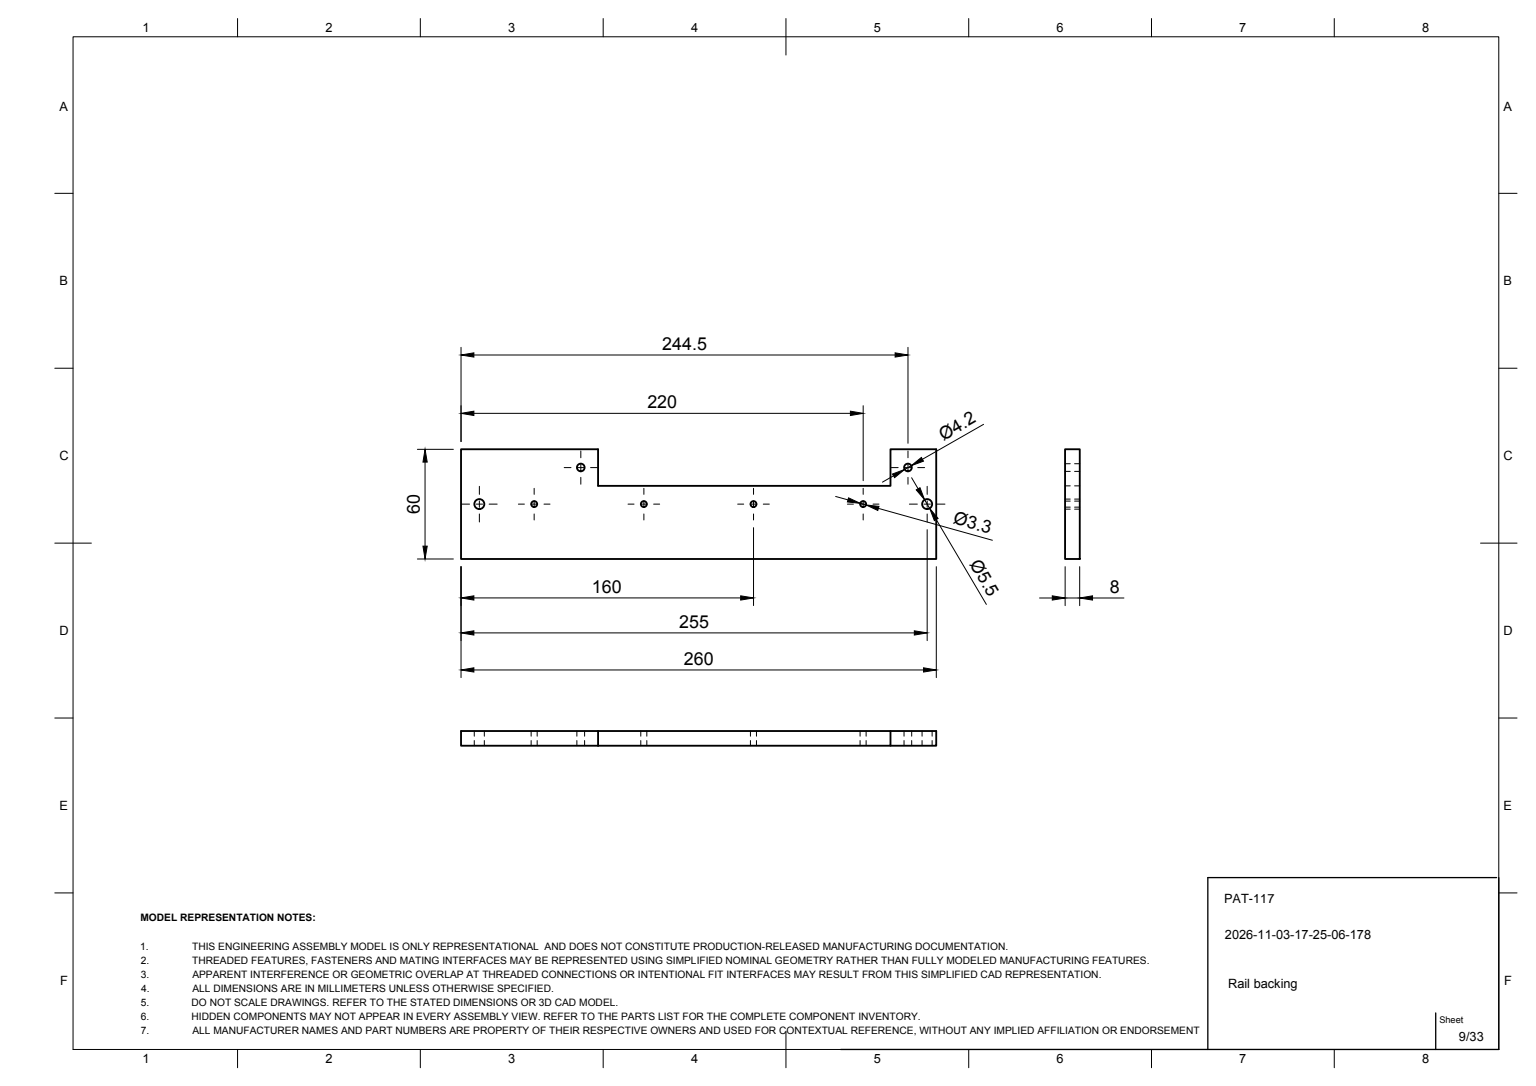
ISO-10303-21;
HEADER;
/* Generated by software containing ST-Developer
 * from STEP Tools, Inc. (www.steptools.com) 
 */

FILE_DESCRIPTION(
/* description */ ('Counterbalanced vertical column'),
/* implementation_level */ '2;1');

FILE_NAME(
/* name */ 'Rail backing.step',
/* time_stamp */ '2026-10-29T16:47:22-07:00',
/* author */ (''),
/* organization */ (''),
/* preprocessor_version */ 'ST-DEVELOPER v20.2',
/* originating_system */ 'Autodesk Translation Framework v15.17.0.0',
/* authorisation */ '');

FILE_SCHEMA (('AUTOMOTIVE_DESIGN { 1 0 10303 214 3 1 1 }'));
ENDSEC;

DATA;
#10=MECHANICAL_DESIGN_GEOMETRIC_PRESENTATION_REPRESENTATION('',(#354),#15040);
#284=SHAPE_REPRESENTATION_RELATIONSHIP('SRR','None',#15188,#319);
#319=ADVANCED_BREP_SHAPE_REPRESENTATION('',(#389),#15007);
#354=STYLED_ITEM('',(#15443),#389);
#389=MANIFOLD_SOLID_BREP('Body1',#7077);
#424=FACE_BOUND('',#1285,.T.);
#425=FACE_BOUND('',#1286,.T.);
#426=FACE_BOUND('',#1287,.T.);
#427=FACE_BOUND('',#1288,.T.);
#428=FACE_BOUND('',#1289,.T.);
#429=FACE_BOUND('',#1290,.T.);
#430=FACE_BOUND('',#1291,.T.);
#431=FACE_BOUND('',#1292,.T.);
#432=FACE_BOUND('',#1296,.T.);
#433=FACE_BOUND('',#1297,.T.);
#434=FACE_BOUND('',#1298,.T.);
#435=FACE_BOUND('',#1299,.T.);
#436=FACE_BOUND('',#1300,.T.);
#437=FACE_BOUND('',#1301,.T.);
#438=FACE_BOUND('',#1302,.T.);
#439=FACE_BOUND('',#1303,.T.);
#559=PLANE('',#7575);
#560=PLANE('',#7576);
#561=PLANE('',#7577);
#562=PLANE('',#7578);
#563=PLANE('',#7579);
#564=PLANE('',#7580);
#565=PLANE('',#7581);
#566=PLANE('',#7582);
#567=PLANE('',#7583);
#568=PLANE('',#7584);
#860=FACE_OUTER_BOUND('',#1273,.T.);
#861=FACE_OUTER_BOUND('',#1274,.T.);
#862=FACE_OUTER_BOUND('',#1275,.T.);
#863=FACE_OUTER_BOUND('',#1276,.T.);
#864=FACE_OUTER_BOUND('',#1277,.T.);
#865=FACE_OUTER_BOUND('',#1278,.T.);
#866=FACE_OUTER_BOUND('',#1279,.T.);
#867=FACE_OUTER_BOUND('',#1280,.T.);
#868=FACE_OUTER_BOUND('',#1281,.T.);
#869=FACE_OUTER_BOUND('',#1282,.T.);
#870=FACE_OUTER_BOUND('',#1283,.T.);
#871=FACE_OUTER_BOUND('',#1284,.T.);
#872=FACE_OUTER_BOUND('',#1293,.T.);
#873=FACE_OUTER_BOUND('',#1294,.T.);
#874=FACE_OUTER_BOUND('',#1295,.T.);
#875=FACE_OUTER_BOUND('',#1304,.T.);
#876=FACE_OUTER_BOUND('',#1305,.T.);
#877=FACE_OUTER_BOUND('',#1306,.T.);
#1273=EDGE_LOOP('',(#4920,#4921,#4922,#4923));
#1274=EDGE_LOOP('',(#4924,#4925,#4926,#4927));
#1275=EDGE_LOOP('',(#4928,#4929,#4930,#4931));
#1276=EDGE_LOOP('',(#4932,#4933,#4934,#4935));
#1277=EDGE_LOOP('',(#4936,#4937,#4938,#4939));
#1278=EDGE_LOOP('',(#4940,#4941,#4942,#4943));
#1279=EDGE_LOOP('',(#4944,#4945,#4946,#4947));
#1280=EDGE_LOOP('',(#4948,#4949,#4950,#4951));
#1281=EDGE_LOOP('',(#4952,#4953,#4954,#4955));
#1282=EDGE_LOOP('',(#4956,#4957,#4958,#4959));
#1283=EDGE_LOOP('',(#4960,#4961,#4962,#4963));
#1284=EDGE_LOOP('',(#4964,#4965,#4966,#4967,#4968,#4969,#4970,#4971));
#1285=EDGE_LOOP('',(#4972));
#1286=EDGE_LOOP('',(#4973));
#1287=EDGE_LOOP('',(#4974));
#1288=EDGE_LOOP('',(#4975));
#1289=EDGE_LOOP('',(#4976));
#1290=EDGE_LOOP('',(#4977));
#1291=EDGE_LOOP('',(#4978));
#1292=EDGE_LOOP('',(#4979));
#1293=EDGE_LOOP('',(#4980,#4981,#4982,#4983));
#1294=EDGE_LOOP('',(#4984,#4985,#4986,#4987));
#1295=EDGE_LOOP('',(#4988,#4989,#4990,#4991,#4992,#4993,#4994,#4995));
#1296=EDGE_LOOP('',(#4996));
#1297=EDGE_LOOP('',(#4997));
#1298=EDGE_LOOP('',(#4998));
#1299=EDGE_LOOP('',(#4999));
#1300=EDGE_LOOP('',(#5000));
#1301=EDGE_LOOP('',(#5001));
#1302=EDGE_LOOP('',(#5002));
#1303=EDGE_LOOP('',(#5003));
#1304=EDGE_LOOP('',(#5004,#5005,#5006,#5007));
#1305=EDGE_LOOP('',(#5008,#5009,#5010,#5011));
#1306=EDGE_LOOP('',(#5012,#5013,#5014,#5015));
#1805=LINE('',#10493,#2476);
#1806=LINE('',#10499,#2477);
#1807=LINE('',#10505,#2478);
#1808=LINE('',#10511,#2479);
#1809=LINE('',#10517,#2480);
#1810=LINE('',#10523,#2481);
#1811=LINE('',#10529,#2482);
#1812=LINE('',#10535,#2483);
#1813=LINE('',#10540,#2484);
#1814=LINE('',#10542,#2485);
#1815=LINE('',#10544,#2486);
#1816=LINE('',#10545,#2487);
#1817=LINE('',#10549,#2488);
#1818=LINE('',#10551,#2489);
#1819=LINE('',#10553,#2490);
#1820=LINE('',#10554,#2491);
#1821=LINE('',#10556,#2492);
#1822=LINE('',#10557,#2493);
#1823=LINE('',#10560,#2494);
#1824=LINE('',#10562,#2495);
#1825=LINE('',#10564,#2496);
#1826=LINE('',#10566,#2497);
#1827=LINE('',#10567,#2498);
#1828=LINE('',#10570,#2499);
#1829=LINE('',#10571,#2500);
#1830=LINE('',#10574,#2501);
#1831=LINE('',#10575,#2502);
#1832=LINE('',#10578,#2503);
#1833=LINE('',#10580,#2504);
#1834=LINE('',#10581,#2505);
#1835=LINE('',#10583,#2506);
#1836=LINE('',#10584,#2507);
#2476=VECTOR('',#8385,0.210000000000001);
#2477=VECTOR('',#8392,0.210000000000001);
#2478=VECTOR('',#8399,0.164999999999999);
#2479=VECTOR('',#8406,0.164999999999999);
#2480=VECTOR('',#8413,0.164999999999999);
#2481=VECTOR('',#8420,0.164999999999999);
#2482=VECTOR('',#8427,0.274999999999999);
#2483=VECTOR('',#8434,0.275);
#2484=VECTOR('',#8439,1.);
#2485=VECTOR('',#8440,1.);
#2486=VECTOR('',#8441,1.);
#2487=VECTOR('',#8442,1.);
#2488=VECTOR('',#8445,1.);
#2489=VECTOR('',#8446,1.);
#2490=VECTOR('',#8447,1.);
#2491=VECTOR('',#8448,1.);
#2492=VECTOR('',#8451,1.);
#2493=VECTOR('',#8452,1.);
#2494=VECTOR('',#8455,1.);
#2495=VECTOR('',#8456,1.);
#2496=VECTOR('',#8457,1.);
#2497=VECTOR('',#8458,1.);
#2498=VECTOR('',#8459,1.);
#2499=VECTOR('',#8462,1.);
#2500=VECTOR('',#8463,1.);
#2501=VECTOR('',#8466,1.);
#2502=VECTOR('',#8467,1.);
#2503=VECTOR('',#8470,1.);
#2504=VECTOR('',#8471,1.);
#2505=VECTOR('',#8472,1.);
#2506=VECTOR('',#8475,1.);
#2507=VECTOR('',#8476,1.);
#3105=CIRCLE('',#7552,0.210000000000001);
#3106=CIRCLE('',#7553,0.210000000000001);
#3107=CIRCLE('',#7555,0.210000000000001);
#3108=CIRCLE('',#7556,0.210000000000001);
#3109=CIRCLE('',#7558,0.164999999999999);
#3110=CIRCLE('',#7559,0.164999999999999);
#3111=CIRCLE('',#7561,0.164999999999999);
#3112=CIRCLE('',#7562,0.164999999999999);
#3113=CIRCLE('',#7564,0.164999999999999);
#3114=CIRCLE('',#7565,0.164999999999999);
#3115=CIRCLE('',#7567,0.164999999999999);
#3116=CIRCLE('',#7568,0.164999999999999);
#3117=CIRCLE('',#7570,0.274999999999999);
#3118=CIRCLE('',#7571,0.274999999999999);
#3119=CIRCLE('',#7573,0.275);
#3120=CIRCLE('',#7574,0.275);
#3350=VERTEX_POINT('',#10490);
#3351=VERTEX_POINT('',#10492);
#3352=VERTEX_POINT('',#10496);
#3353=VERTEX_POINT('',#10498);
#3354=VERTEX_POINT('',#10502);
#3355=VERTEX_POINT('',#10504);
#3356=VERTEX_POINT('',#10508);
#3357=VERTEX_POINT('',#10510);
#3358=VERTEX_POINT('',#10514);
#3359=VERTEX_POINT('',#10516);
#3360=VERTEX_POINT('',#10520);
#3361=VERTEX_POINT('',#10522);
#3362=VERTEX_POINT('',#10526);
#3363=VERTEX_POINT('',#10528);
#3364=VERTEX_POINT('',#10532);
#3365=VERTEX_POINT('',#10534);
#3366=VERTEX_POINT('',#10538);
#3367=VERTEX_POINT('',#10539);
#3368=VERTEX_POINT('',#10541);
#3369=VERTEX_POINT('',#10543);
#3370=VERTEX_POINT('',#10547);
#3371=VERTEX_POINT('',#10548);
#3372=VERTEX_POINT('',#10550);
#3373=VERTEX_POINT('',#10552);
#3374=VERTEX_POINT('',#10559);
#3375=VERTEX_POINT('',#10561);
#3376=VERTEX_POINT('',#10563);
#3377=VERTEX_POINT('',#10565);
#3378=VERTEX_POINT('',#10569);
#3379=VERTEX_POINT('',#10573);
#3380=VERTEX_POINT('',#10577);
#3381=VERTEX_POINT('',#10579);
#3961=EDGE_CURVE('',#3350,#3350,#3105,.T.);
#3962=EDGE_CURVE('',#3350,#3351,#1805,.T.);
#3963=EDGE_CURVE('',#3351,#3351,#3106,.T.);
#3964=EDGE_CURVE('',#3352,#3352,#3107,.T.);
#3965=EDGE_CURVE('',#3352,#3353,#1806,.T.);
#3966=EDGE_CURVE('',#3353,#3353,#3108,.T.);
#3967=EDGE_CURVE('',#3354,#3354,#3109,.T.);
#3968=EDGE_CURVE('',#3354,#3355,#1807,.T.);
#3969=EDGE_CURVE('',#3355,#3355,#3110,.T.);
#3970=EDGE_CURVE('',#3356,#3356,#3111,.T.);
#3971=EDGE_CURVE('',#3356,#3357,#1808,.T.);
#3972=EDGE_CURVE('',#3357,#3357,#3112,.T.);
#3973=EDGE_CURVE('',#3358,#3358,#3113,.T.);
#3974=EDGE_CURVE('',#3358,#3359,#1809,.T.);
#3975=EDGE_CURVE('',#3359,#3359,#3114,.T.);
#3976=EDGE_CURVE('',#3360,#3360,#3115,.T.);
#3977=EDGE_CURVE('',#3360,#3361,#1810,.T.);
#3978=EDGE_CURVE('',#3361,#3361,#3116,.T.);
#3979=EDGE_CURVE('',#3362,#3362,#3117,.T.);
#3980=EDGE_CURVE('',#3362,#3363,#1811,.T.);
#3981=EDGE_CURVE('',#3363,#3363,#3118,.T.);
#3982=EDGE_CURVE('',#3364,#3364,#3119,.T.);
#3983=EDGE_CURVE('',#3364,#3365,#1812,.T.);
#3984=EDGE_CURVE('',#3365,#3365,#3120,.T.);
#3985=EDGE_CURVE('',#3366,#3367,#1813,.T.);
#3986=EDGE_CURVE('',#3368,#3366,#1814,.T.);
#3987=EDGE_CURVE('',#3369,#3368,#1815,.T.);
#3988=EDGE_CURVE('',#3367,#3369,#1816,.T.);
#3989=EDGE_CURVE('',#3370,#3371,#1817,.T.);
#3990=EDGE_CURVE('',#3372,#3370,#1818,.T.);
#3991=EDGE_CURVE('',#3373,#3372,#1819,.T.);
#3992=EDGE_CURVE('',#3373,#3371,#1820,.T.);
#3993=EDGE_CURVE('',#3371,#3366,#1821,.T.);
#3994=EDGE_CURVE('',#3368,#3373,#1822,.T.);
#3995=EDGE_CURVE('',#3374,#3372,#1823,.T.);
#3996=EDGE_CURVE('',#3374,#3375,#1824,.T.);
#3997=EDGE_CURVE('',#3375,#3376,#1825,.T.);
#3998=EDGE_CURVE('',#3377,#3376,#1826,.T.);
#3999=EDGE_CURVE('',#3369,#3377,#1827,.T.);
#4000=EDGE_CURVE('',#3378,#3370,#1828,.T.);
#4001=EDGE_CURVE('',#3378,#3374,#1829,.T.);
#4002=EDGE_CURVE('',#3379,#3377,#1830,.T.);
#4003=EDGE_CURVE('',#3367,#3379,#1831,.T.);
#4004=EDGE_CURVE('',#3380,#3379,#1832,.T.);
#4005=EDGE_CURVE('',#3381,#3380,#1833,.T.);
#4006=EDGE_CURVE('',#3381,#3378,#1834,.T.);
#4007=EDGE_CURVE('',#3375,#3381,#1835,.T.);
#4008=EDGE_CURVE('',#3376,#3380,#1836,.T.);
#4920=ORIENTED_EDGE('',*,*,#3961,.F.);
#4921=ORIENTED_EDGE('',*,*,#3962,.T.);
#4922=ORIENTED_EDGE('',*,*,#3963,.F.);
#4923=ORIENTED_EDGE('',*,*,#3962,.F.);
#4924=ORIENTED_EDGE('',*,*,#3964,.F.);
#4925=ORIENTED_EDGE('',*,*,#3965,.T.);
#4926=ORIENTED_EDGE('',*,*,#3966,.F.);
#4927=ORIENTED_EDGE('',*,*,#3965,.F.);
#4928=ORIENTED_EDGE('',*,*,#3967,.F.);
#4929=ORIENTED_EDGE('',*,*,#3968,.T.);
#4930=ORIENTED_EDGE('',*,*,#3969,.F.);
#4931=ORIENTED_EDGE('',*,*,#3968,.F.);
#4932=ORIENTED_EDGE('',*,*,#3970,.F.);
#4933=ORIENTED_EDGE('',*,*,#3971,.T.);
#4934=ORIENTED_EDGE('',*,*,#3972,.F.);
#4935=ORIENTED_EDGE('',*,*,#3971,.F.);
#4936=ORIENTED_EDGE('',*,*,#3973,.F.);
#4937=ORIENTED_EDGE('',*,*,#3974,.T.);
#4938=ORIENTED_EDGE('',*,*,#3975,.F.);
#4939=ORIENTED_EDGE('',*,*,#3974,.F.);
#4940=ORIENTED_EDGE('',*,*,#3976,.F.);
#4941=ORIENTED_EDGE('',*,*,#3977,.T.);
#4942=ORIENTED_EDGE('',*,*,#3978,.F.);
#4943=ORIENTED_EDGE('',*,*,#3977,.F.);
#4944=ORIENTED_EDGE('',*,*,#3979,.F.);
#4945=ORIENTED_EDGE('',*,*,#3980,.T.);
#4946=ORIENTED_EDGE('',*,*,#3981,.F.);
#4947=ORIENTED_EDGE('',*,*,#3980,.F.);
#4948=ORIENTED_EDGE('',*,*,#3982,.F.);
#4949=ORIENTED_EDGE('',*,*,#3983,.T.);
#4950=ORIENTED_EDGE('',*,*,#3984,.F.);
#4951=ORIENTED_EDGE('',*,*,#3983,.F.);
#4952=ORIENTED_EDGE('',*,*,#3985,.F.);
#4953=ORIENTED_EDGE('',*,*,#3986,.F.);
#4954=ORIENTED_EDGE('',*,*,#3987,.F.);
#4955=ORIENTED_EDGE('',*,*,#3988,.F.);
#4956=ORIENTED_EDGE('',*,*,#3989,.F.);
#4957=ORIENTED_EDGE('',*,*,#3990,.F.);
#4958=ORIENTED_EDGE('',*,*,#3991,.F.);
#4959=ORIENTED_EDGE('',*,*,#3992,.T.);
#4960=ORIENTED_EDGE('',*,*,#3993,.F.);
#4961=ORIENTED_EDGE('',*,*,#3992,.F.);
#4962=ORIENTED_EDGE('',*,*,#3994,.F.);
#4963=ORIENTED_EDGE('',*,*,#3986,.T.);
#4964=ORIENTED_EDGE('',*,*,#3987,.T.);
#4965=ORIENTED_EDGE('',*,*,#3994,.T.);
#4966=ORIENTED_EDGE('',*,*,#3991,.T.);
#4967=ORIENTED_EDGE('',*,*,#3995,.F.);
#4968=ORIENTED_EDGE('',*,*,#3996,.T.);
#4969=ORIENTED_EDGE('',*,*,#3997,.T.);
#4970=ORIENTED_EDGE('',*,*,#3998,.F.);
#4971=ORIENTED_EDGE('',*,*,#3999,.F.);
#4972=ORIENTED_EDGE('',*,*,#3982,.T.);
#4973=ORIENTED_EDGE('',*,*,#3979,.T.);
#4974=ORIENTED_EDGE('',*,*,#3976,.T.);
#4975=ORIENTED_EDGE('',*,*,#3973,.T.);
#4976=ORIENTED_EDGE('',*,*,#3970,.T.);
#4977=ORIENTED_EDGE('',*,*,#3967,.T.);
#4978=ORIENTED_EDGE('',*,*,#3964,.T.);
#4979=ORIENTED_EDGE('',*,*,#3961,.T.);
#4980=ORIENTED_EDGE('',*,*,#3990,.T.);
#4981=ORIENTED_EDGE('',*,*,#4000,.F.);
#4982=ORIENTED_EDGE('',*,*,#4001,.T.);
#4983=ORIENTED_EDGE('',*,*,#3995,.T.);
#4984=ORIENTED_EDGE('',*,*,#3988,.T.);
#4985=ORIENTED_EDGE('',*,*,#3999,.T.);
#4986=ORIENTED_EDGE('',*,*,#4002,.F.);
#4987=ORIENTED_EDGE('',*,*,#4003,.F.);
#4988=ORIENTED_EDGE('',*,*,#3985,.T.);
#4989=ORIENTED_EDGE('',*,*,#4003,.T.);
#4990=ORIENTED_EDGE('',*,*,#4004,.F.);
#4991=ORIENTED_EDGE('',*,*,#4005,.F.);
#4992=ORIENTED_EDGE('',*,*,#4006,.T.);
#4993=ORIENTED_EDGE('',*,*,#4000,.T.);
#4994=ORIENTED_EDGE('',*,*,#3989,.T.);
#4995=ORIENTED_EDGE('',*,*,#3993,.T.);
#4996=ORIENTED_EDGE('',*,*,#3984,.T.);
#4997=ORIENTED_EDGE('',*,*,#3981,.T.);
#4998=ORIENTED_EDGE('',*,*,#3978,.T.);
#4999=ORIENTED_EDGE('',*,*,#3975,.T.);
#5000=ORIENTED_EDGE('',*,*,#3972,.T.);
#5001=ORIENTED_EDGE('',*,*,#3969,.T.);
#5002=ORIENTED_EDGE('',*,*,#3966,.T.);
#5003=ORIENTED_EDGE('',*,*,#3963,.T.);
#5004=ORIENTED_EDGE('',*,*,#4007,.T.);
#5005=ORIENTED_EDGE('',*,*,#4005,.T.);
#5006=ORIENTED_EDGE('',*,*,#4008,.F.);
#5007=ORIENTED_EDGE('',*,*,#3997,.F.);
#5008=ORIENTED_EDGE('',*,*,#3998,.T.);
#5009=ORIENTED_EDGE('',*,*,#4008,.T.);
#5010=ORIENTED_EDGE('',*,*,#4004,.T.);
#5011=ORIENTED_EDGE('',*,*,#4002,.T.);
#5012=ORIENTED_EDGE('',*,*,#3996,.F.);
#5013=ORIENTED_EDGE('',*,*,#4001,.F.);
#5014=ORIENTED_EDGE('',*,*,#4006,.F.);
#5015=ORIENTED_EDGE('',*,*,#4007,.F.);
#6580=CYLINDRICAL_SURFACE('',#7551,0.210000000000001);
#6581=CYLINDRICAL_SURFACE('',#7554,0.210000000000001);
#6582=CYLINDRICAL_SURFACE('',#7557,0.164999999999999);
#6583=CYLINDRICAL_SURFACE('',#7560,0.164999999999999);
#6584=CYLINDRICAL_SURFACE('',#7563,0.164999999999999);
#6585=CYLINDRICAL_SURFACE('',#7566,0.164999999999999);
#6586=CYLINDRICAL_SURFACE('',#7569,0.274999999999999);
#6587=CYLINDRICAL_SURFACE('',#7572,0.275);
#6702=ADVANCED_FACE('',(#860),#6580,.F.);
#6703=ADVANCED_FACE('',(#861),#6581,.F.);
#6704=ADVANCED_FACE('',(#862),#6582,.F.);
#6705=ADVANCED_FACE('',(#863),#6583,.F.);
#6706=ADVANCED_FACE('',(#864),#6584,.F.);
#6707=ADVANCED_FACE('',(#865),#6585,.F.);
#6708=ADVANCED_FACE('',(#866),#6586,.F.);
#6709=ADVANCED_FACE('',(#867),#6587,.F.);
#6710=ADVANCED_FACE('',(#868),#559,.F.);
#6711=ADVANCED_FACE('',(#869),#560,.F.);
#6712=ADVANCED_FACE('',(#870),#561,.F.);
#6713=ADVANCED_FACE('',(#871,#424,#425,#426,#427,#428,#429,#430,#431),#562,
 .T.);
#6714=ADVANCED_FACE('',(#872),#563,.T.);
#6715=ADVANCED_FACE('',(#873),#564,.T.);
#6716=ADVANCED_FACE('',(#874,#432,#433,#434,#435,#436,#437,#438,#439),#565,
 .T.);
#6717=ADVANCED_FACE('',(#875),#566,.T.);
#6718=ADVANCED_FACE('',(#876),#567,.T.);
#6719=ADVANCED_FACE('',(#877),#568,.F.);
#7077=CLOSED_SHELL('',(#6702,#6703,#6704,#6705,#6706,#6707,#6708,#6709,
#6710,#6711,#6712,#6713,#6714,#6715,#6716,#6717,#6718,#6719));
#7550=AXIS2_PLACEMENT_3D('',#10488,#8379,#8380);
#7551=AXIS2_PLACEMENT_3D('',#10489,#8381,#8382);
#7552=AXIS2_PLACEMENT_3D('',#10491,#8383,#8384);
#7553=AXIS2_PLACEMENT_3D('',#10494,#8386,#8387);
#7554=AXIS2_PLACEMENT_3D('',#10495,#8388,#8389);
#7555=AXIS2_PLACEMENT_3D('',#10497,#8390,#8391);
#7556=AXIS2_PLACEMENT_3D('',#10500,#8393,#8394);
#7557=AXIS2_PLACEMENT_3D('',#10501,#8395,#8396);
#7558=AXIS2_PLACEMENT_3D('',#10503,#8397,#8398);
#7559=AXIS2_PLACEMENT_3D('',#10506,#8400,#8401);
#7560=AXIS2_PLACEMENT_3D('',#10507,#8402,#8403);
#7561=AXIS2_PLACEMENT_3D('',#10509,#8404,#8405);
#7562=AXIS2_PLACEMENT_3D('',#10512,#8407,#8408);
#7563=AXIS2_PLACEMENT_3D('',#10513,#8409,#8410);
#7564=AXIS2_PLACEMENT_3D('',#10515,#8411,#8412);
#7565=AXIS2_PLACEMENT_3D('',#10518,#8414,#8415);
#7566=AXIS2_PLACEMENT_3D('',#10519,#8416,#8417);
#7567=AXIS2_PLACEMENT_3D('',#10521,#8418,#8419);
#7568=AXIS2_PLACEMENT_3D('',#10524,#8421,#8422);
#7569=AXIS2_PLACEMENT_3D('',#10525,#8423,#8424);
#7570=AXIS2_PLACEMENT_3D('',#10527,#8425,#8426);
#7571=AXIS2_PLACEMENT_3D('',#10530,#8428,#8429);
#7572=AXIS2_PLACEMENT_3D('',#10531,#8430,#8431);
#7573=AXIS2_PLACEMENT_3D('',#10533,#8432,#8433);
#7574=AXIS2_PLACEMENT_3D('',#10536,#8435,#8436);
#7575=AXIS2_PLACEMENT_3D('',#10537,#8437,#8438);
#7576=AXIS2_PLACEMENT_3D('',#10546,#8443,#8444);
#7577=AXIS2_PLACEMENT_3D('',#10555,#8449,#8450);
#7578=AXIS2_PLACEMENT_3D('',#10558,#8453,#8454);
#7579=AXIS2_PLACEMENT_3D('',#10568,#8460,#8461);
#7580=AXIS2_PLACEMENT_3D('',#10572,#8464,#8465);
#7581=AXIS2_PLACEMENT_3D('',#10576,#8468,#8469);
#7582=AXIS2_PLACEMENT_3D('',#10582,#8473,#8474);
#7583=AXIS2_PLACEMENT_3D('',#10585,#8477,#8478);
#7584=AXIS2_PLACEMENT_3D('',#10586,#8479,#8480);
#8379=DIRECTION('axis',(0.,0.,1.));
#8380=DIRECTION('refdir',(1.,0.,0.));
#8381=DIRECTION('center_axis',(1.,0.,0.));
#8382=DIRECTION('ref_axis',(0.,0.,-1.));
#8383=DIRECTION('center_axis',(1.,0.,0.));
#8384=DIRECTION('ref_axis',(0.,0.,-1.));
#8385=DIRECTION('',(1.,0.,0.));
#8386=DIRECTION('center_axis',(-1.,0.,0.));
#8387=DIRECTION('ref_axis',(0.,0.,-1.));
#8388=DIRECTION('center_axis',(1.,0.,0.));
#8389=DIRECTION('ref_axis',(0.,0.,-1.));
#8390=DIRECTION('center_axis',(1.,0.,0.));
#8391=DIRECTION('ref_axis',(0.,0.,-1.));
#8392=DIRECTION('',(1.,0.,0.));
#8393=DIRECTION('center_axis',(-1.,0.,0.));
#8394=DIRECTION('ref_axis',(0.,0.,-1.));
#8395=DIRECTION('center_axis',(1.,0.,0.));
#8396=DIRECTION('ref_axis',(0.,0.,-1.));
#8397=DIRECTION('center_axis',(1.,0.,0.));
#8398=DIRECTION('ref_axis',(0.,0.,-1.));
#8399=DIRECTION('',(1.,0.,0.));
#8400=DIRECTION('center_axis',(-1.,0.,0.));
#8401=DIRECTION('ref_axis',(0.,0.,-1.));
#8402=DIRECTION('center_axis',(1.,0.,0.));
#8403=DIRECTION('ref_axis',(0.,0.,-1.));
#8404=DIRECTION('center_axis',(1.,0.,0.));
#8405=DIRECTION('ref_axis',(0.,0.,-1.));
#8406=DIRECTION('',(1.,0.,0.));
#8407=DIRECTION('center_axis',(-1.,0.,0.));
#8408=DIRECTION('ref_axis',(0.,0.,-1.));
#8409=DIRECTION('center_axis',(1.,0.,0.));
#8410=DIRECTION('ref_axis',(0.,0.,-1.));
#8411=DIRECTION('center_axis',(1.,0.,0.));
#8412=DIRECTION('ref_axis',(0.,0.,-1.));
#8413=DIRECTION('',(1.,0.,0.));
#8414=DIRECTION('center_axis',(-1.,0.,0.));
#8415=DIRECTION('ref_axis',(0.,0.,-1.));
#8416=DIRECTION('center_axis',(1.,0.,0.));
#8417=DIRECTION('ref_axis',(0.,0.,-1.));
#8418=DIRECTION('center_axis',(1.,0.,0.));
#8419=DIRECTION('ref_axis',(0.,0.,-1.));
#8420=DIRECTION('',(1.,0.,0.));
#8421=DIRECTION('center_axis',(-1.,0.,0.));
#8422=DIRECTION('ref_axis',(0.,0.,-1.));
#8423=DIRECTION('center_axis',(1.,0.,0.));
#8424=DIRECTION('ref_axis',(0.,0.,-1.));
#8425=DIRECTION('center_axis',(1.,0.,0.));
#8426=DIRECTION('ref_axis',(0.,0.,-1.));
#8427=DIRECTION('',(1.,0.,0.));
#8428=DIRECTION('center_axis',(-1.,0.,0.));
#8429=DIRECTION('ref_axis',(0.,0.,-1.));
#8430=DIRECTION('center_axis',(1.,0.,0.));
#8431=DIRECTION('ref_axis',(0.,0.,-1.));
#8432=DIRECTION('center_axis',(1.,0.,0.));
#8433=DIRECTION('ref_axis',(0.,0.,-1.));
#8434=DIRECTION('',(1.,0.,0.));
#8435=DIRECTION('center_axis',(-1.,0.,0.));
#8436=DIRECTION('ref_axis',(0.,0.,-1.));
#8437=DIRECTION('center_axis',(0.,0.,1.));
#8438=DIRECTION('ref_axis',(0.,-1.,0.));
#8439=DIRECTION('',(0.,1.,0.));
#8440=DIRECTION('',(1.,0.,0.));
#8441=DIRECTION('',(0.,-1.,0.));
#8442=DIRECTION('',(-1.,0.,0.));
#8443=DIRECTION('center_axis',(0.,0.,-1.));
#8444=DIRECTION('ref_axis',(0.,1.,0.));
#8445=DIRECTION('',(0.,-1.,0.));
#8446=DIRECTION('',(1.,0.,0.));
#8447=DIRECTION('',(0.,1.,0.));
#8448=DIRECTION('',(1.,0.,0.));
#8449=DIRECTION('center_axis',(0.,-1.,0.));
#8450=DIRECTION('ref_axis',(0.,0.,-1.));
#8451=DIRECTION('',(0.,0.,1.));
#8452=DIRECTION('',(0.,0.,-1.));
#8453=DIRECTION('center_axis',(-1.,0.,0.));
#8454=DIRECTION('ref_axis',(0.,-1.,0.));
#8455=DIRECTION('',(0.,0.,1.));
#8456=DIRECTION('',(0.,-1.,0.));
#8457=DIRECTION('',(0.,0.,1.));
#8458=DIRECTION('',(0.,-1.,0.));
#8459=DIRECTION('',(0.,0.,1.));
#8460=DIRECTION('center_axis',(0.,1.,0.));
#8461=DIRECTION('ref_axis',(-1.,0.,0.));
#8462=DIRECTION('',(0.,0.,1.));
#8463=DIRECTION('',(-1.,0.,0.));
#8464=DIRECTION('center_axis',(0.,1.,0.));
#8465=DIRECTION('ref_axis',(-1.,0.,0.));
#8466=DIRECTION('',(-1.,0.,0.));
#8467=DIRECTION('',(0.,0.,1.));
#8468=DIRECTION('center_axis',(1.,0.,0.));
#8469=DIRECTION('ref_axis',(0.,1.,0.));
#8470=DIRECTION('',(0.,1.,0.));
#8471=DIRECTION('',(0.,0.,1.));
#8472=DIRECTION('',(0.,1.,0.));
#8473=DIRECTION('center_axis',(0.,-1.,0.));
#8474=DIRECTION('ref_axis',(1.,0.,0.));
#8475=DIRECTION('',(1.,0.,0.));
#8476=DIRECTION('',(1.,0.,0.));
#8477=DIRECTION('center_axis',(0.,0.,1.));
#8478=DIRECTION('ref_axis',(1.,0.,0.));
#8479=DIRECTION('center_axis',(0.,0.,1.));
#8480=DIRECTION('ref_axis',(1.,0.,0.));
#10488=CARTESIAN_POINT('',(0.,0.,0.));
#10489=CARTESIAN_POINT('Origin',(1.1,2.,33.45));
#10490=CARTESIAN_POINT('',(1.2,2.,33.66));
#10491=CARTESIAN_POINT('Origin',(1.2,2.,33.45));
#10492=CARTESIAN_POINT('',(2.,2.,33.66));
#10493=CARTESIAN_POINT('',(1.1,2.,33.66));
#10494=CARTESIAN_POINT('Origin',(2.,2.,33.45));
#10495=CARTESIAN_POINT('Origin',(1.1,2.,15.55));
#10496=CARTESIAN_POINT('',(1.2,2.,15.76));
#10497=CARTESIAN_POINT('Origin',(1.2,2.,15.55));
#10498=CARTESIAN_POINT('',(2.,2.,15.76));
#10499=CARTESIAN_POINT('',(1.1,2.,15.76));
#10500=CARTESIAN_POINT('Origin',(2.,2.,15.55));
#10501=CARTESIAN_POINT('Origin',(1.1,0.,36.));
#10502=CARTESIAN_POINT('',(1.2,-2.02066721859312E-17,36.165));
#10503=CARTESIAN_POINT('Origin',(1.2,0.,36.));
#10504=CARTESIAN_POINT('',(2.,2.02066721859312E-17,36.165));
#10505=CARTESIAN_POINT('',(1.1,-2.02066721859312E-17,36.165));
#10506=CARTESIAN_POINT('Origin',(2.,0.,36.));
#10507=CARTESIAN_POINT('Origin',(1.1,0.,30.));
#10508=CARTESIAN_POINT('',(1.2,-2.02066721859312E-17,30.165));
#10509=CARTESIAN_POINT('Origin',(1.2,0.,30.));
#10510=CARTESIAN_POINT('',(2.,2.02066721859312E-17,30.165));
#10511=CARTESIAN_POINT('',(1.1,-2.02066721859312E-17,30.165));
#10512=CARTESIAN_POINT('Origin',(2.,0.,30.));
#10513=CARTESIAN_POINT('Origin',(1.1,0.,24.));
#10514=CARTESIAN_POINT('',(1.2,-2.02066721859312E-17,24.165));
#10515=CARTESIAN_POINT('Origin',(1.2,0.,24.));
#10516=CARTESIAN_POINT('',(2.,2.02066721859312E-17,24.165));
#10517=CARTESIAN_POINT('',(1.1,-2.02066721859312E-17,24.165));
#10518=CARTESIAN_POINT('Origin',(2.,0.,24.));
#10519=CARTESIAN_POINT('Origin',(1.1,0.,18.));
#10520=CARTESIAN_POINT('',(1.2,-2.02066721859312E-17,18.165));
#10521=CARTESIAN_POINT('Origin',(1.2,0.,18.));
#10522=CARTESIAN_POINT('',(2.,2.02066721859312E-17,18.165));
#10523=CARTESIAN_POINT('',(1.1,-2.02066721859312E-17,18.165));
#10524=CARTESIAN_POINT('Origin',(2.,0.,18.));
#10525=CARTESIAN_POINT('Origin',(1.1,0.,39.));
#10526=CARTESIAN_POINT('',(1.2,-3.3677786976552E-17,39.275));
#10527=CARTESIAN_POINT('Origin',(1.2,0.,39.));
#10528=CARTESIAN_POINT('',(2.,3.3677786976552E-17,39.275));
#10529=CARTESIAN_POINT('',(1.1,-3.3677786976552E-17,39.275));
#10530=CARTESIAN_POINT('Origin',(2.,0.,39.));
#10531=CARTESIAN_POINT('Origin',(1.1,0.,14.5));
#10532=CARTESIAN_POINT('',(1.2,-3.36777869765523E-17,14.775));
#10533=CARTESIAN_POINT('Origin',(1.2,0.,14.5));
#10534=CARTESIAN_POINT('',(2.,3.36777869765523E-17,14.775));
#10535=CARTESIAN_POINT('',(1.1,-3.36777869765523E-17,14.775));
#10536=CARTESIAN_POINT('Origin',(2.,0.,14.5));
#10537=CARTESIAN_POINT('Origin',(1.1,3.1,32.5));
#10538=CARTESIAN_POINT('',(2.,1.,32.5));
#10539=CARTESIAN_POINT('',(2.,3.,32.5));
#10540=CARTESIAN_POINT('',(2.,0.05,32.5));
#10541=CARTESIAN_POINT('',(1.2,1.,32.5));
#10542=CARTESIAN_POINT('',(1.1,1.,32.5));
#10543=CARTESIAN_POINT('',(1.2,3.,32.5));
#10544=CARTESIAN_POINT('',(1.2,3.05,32.5));
#10545=CARTESIAN_POINT('',(1.55,3.,32.5));
#10546=CARTESIAN_POINT('Origin',(1.1,1.,16.5));
#10547=CARTESIAN_POINT('',(2.,3.,16.5));
#10548=CARTESIAN_POINT('',(2.,1.,16.5));
#10549=CARTESIAN_POINT('',(2.,-1.,16.5));
#10550=CARTESIAN_POINT('',(1.2,3.,16.5));
#10551=CARTESIAN_POINT('',(1.55,3.,16.5));
#10552=CARTESIAN_POINT('',(1.2,1.,16.5));
#10553=CARTESIAN_POINT('',(1.2,2.,16.5));
#10554=CARTESIAN_POINT('',(1.1,1.,16.5));
#10555=CARTESIAN_POINT('Origin',(1.1,1.,32.5));
#10556=CARTESIAN_POINT('',(2.,1.,23.25));
#10557=CARTESIAN_POINT('',(1.2,1.,23.25));
#10558=CARTESIAN_POINT('Origin',(1.2,3.,14.));
#10559=CARTESIAN_POINT('',(1.2,3.,14.));
#10560=CARTESIAN_POINT('',(1.2,3.,14.));
#10561=CARTESIAN_POINT('',(1.2,-3.,14.));
#10562=CARTESIAN_POINT('',(1.2,3.,14.));
#10563=CARTESIAN_POINT('',(1.2,-3.,40.));
#10564=CARTESIAN_POINT('',(1.2,-3.,14.));
#10565=CARTESIAN_POINT('',(1.2,3.,40.));
#10566=CARTESIAN_POINT('',(1.2,3.,40.));
#10567=CARTESIAN_POINT('',(1.2,3.,14.));
#10568=CARTESIAN_POINT('Origin',(2.,3.,14.));
#10569=CARTESIAN_POINT('',(2.,3.,14.));
#10570=CARTESIAN_POINT('',(2.,3.,14.));
#10571=CARTESIAN_POINT('',(2.,3.,14.));
#10572=CARTESIAN_POINT('Origin',(2.,3.,14.));
#10573=CARTESIAN_POINT('',(2.,3.,40.));
#10574=CARTESIAN_POINT('',(2.,3.,40.));
#10575=CARTESIAN_POINT('',(2.,3.,14.));
#10576=CARTESIAN_POINT('Origin',(2.,-3.,14.));
#10577=CARTESIAN_POINT('',(2.,-3.,40.));
#10578=CARTESIAN_POINT('',(2.,-3.,40.));
#10579=CARTESIAN_POINT('',(2.,-3.,14.));
#10580=CARTESIAN_POINT('',(2.,-3.,14.));
#10581=CARTESIAN_POINT('',(2.,-3.,14.));
#10582=CARTESIAN_POINT('Origin',(1.2,-3.,14.));
#10583=CARTESIAN_POINT('',(1.2,-3.,14.));
#10584=CARTESIAN_POINT('',(1.2,-3.,40.));
#10585=CARTESIAN_POINT('Origin',(1.6,0.,40.));
#10586=CARTESIAN_POINT('Origin',(1.6,0.,14.));
#14967=UNCERTAINTY_MEASURE_WITH_UNIT(LENGTH_MEASURE(0.001),#15041,
'DISTANCE_ACCURACY_VALUE',
'Maximum model space distance between geometric entities at asserted c
onnectivities');
#15000=UNCERTAINTY_MEASURE_WITH_UNIT(LENGTH_MEASURE(0.001),#15041,
'DISTANCE_ACCURACY_VALUE',
'Maximum model space distance between geometric entities at asserted c
onnectivities');
#15007=(
GEOMETRIC_REPRESENTATION_CONTEXT(3)
GLOBAL_UNCERTAINTY_ASSIGNED_CONTEXT((#14967))
GLOBAL_UNIT_ASSIGNED_CONTEXT((#15041,#15043,#15044))
REPRESENTATION_CONTEXT('','3D')
);
#15040=(
GEOMETRIC_REPRESENTATION_CONTEXT(3)
GLOBAL_UNCERTAINTY_ASSIGNED_CONTEXT((#15000))
GLOBAL_UNIT_ASSIGNED_CONTEXT((#15041,#15043,#15044))
REPRESENTATION_CONTEXT('','3D')
);
#15041=(
LENGTH_UNIT()
NAMED_UNIT(*)
SI_UNIT(.CENTI.,.METRE.)
);
#15043=(
NAMED_UNIT(*)
PLANE_ANGLE_UNIT()
SI_UNIT($,.RADIAN.)
);
#15044=(
NAMED_UNIT(*)
SI_UNIT($,.STERADIAN.)
SOLID_ANGLE_UNIT()
);
#15051=SHAPE_DEFINITION_REPRESENTATION(#15090,#15188);
#15090=PRODUCT_DEFINITION_SHAPE('',$,#15228);
#15188=SHAPE_REPRESENTATION('',(#7550),#15007);
#15221=PRODUCT_DEFINITION_CONTEXT('part definition',#15340,'design');
#15228=PRODUCT_DEFINITION('Rail backing','Rail backing',#15267,#15221);
#15267=PRODUCT_DEFINITION_FORMATION('',$,#15348);
#15340=APPLICATION_CONTEXT(
'Core Data for Automotive Mechanical Design Process');
#15341=PRODUCT_CONTEXT('part definition',#15340,'mechanical');
#15348=PRODUCT('Rail backing','Rail backing','Rail backing',(#15341));
#15437=COLOUR_RGB('Light Blue',0.38,0.62,0.78);
#15438=FILL_AREA_STYLE_COLOUR('',#15437);
#15439=FILL_AREA_STYLE('',(#15438));
#15440=SURFACE_STYLE_FILL_AREA(#15439);
#15441=SURFACE_SIDE_STYLE('',(#15440));
#15442=SURFACE_STYLE_USAGE(.BOTH.,#15441);
#15443=PRESENTATION_STYLE_ASSIGNMENT((#15442));
ENDSEC;
END-ISO-10303-21;
